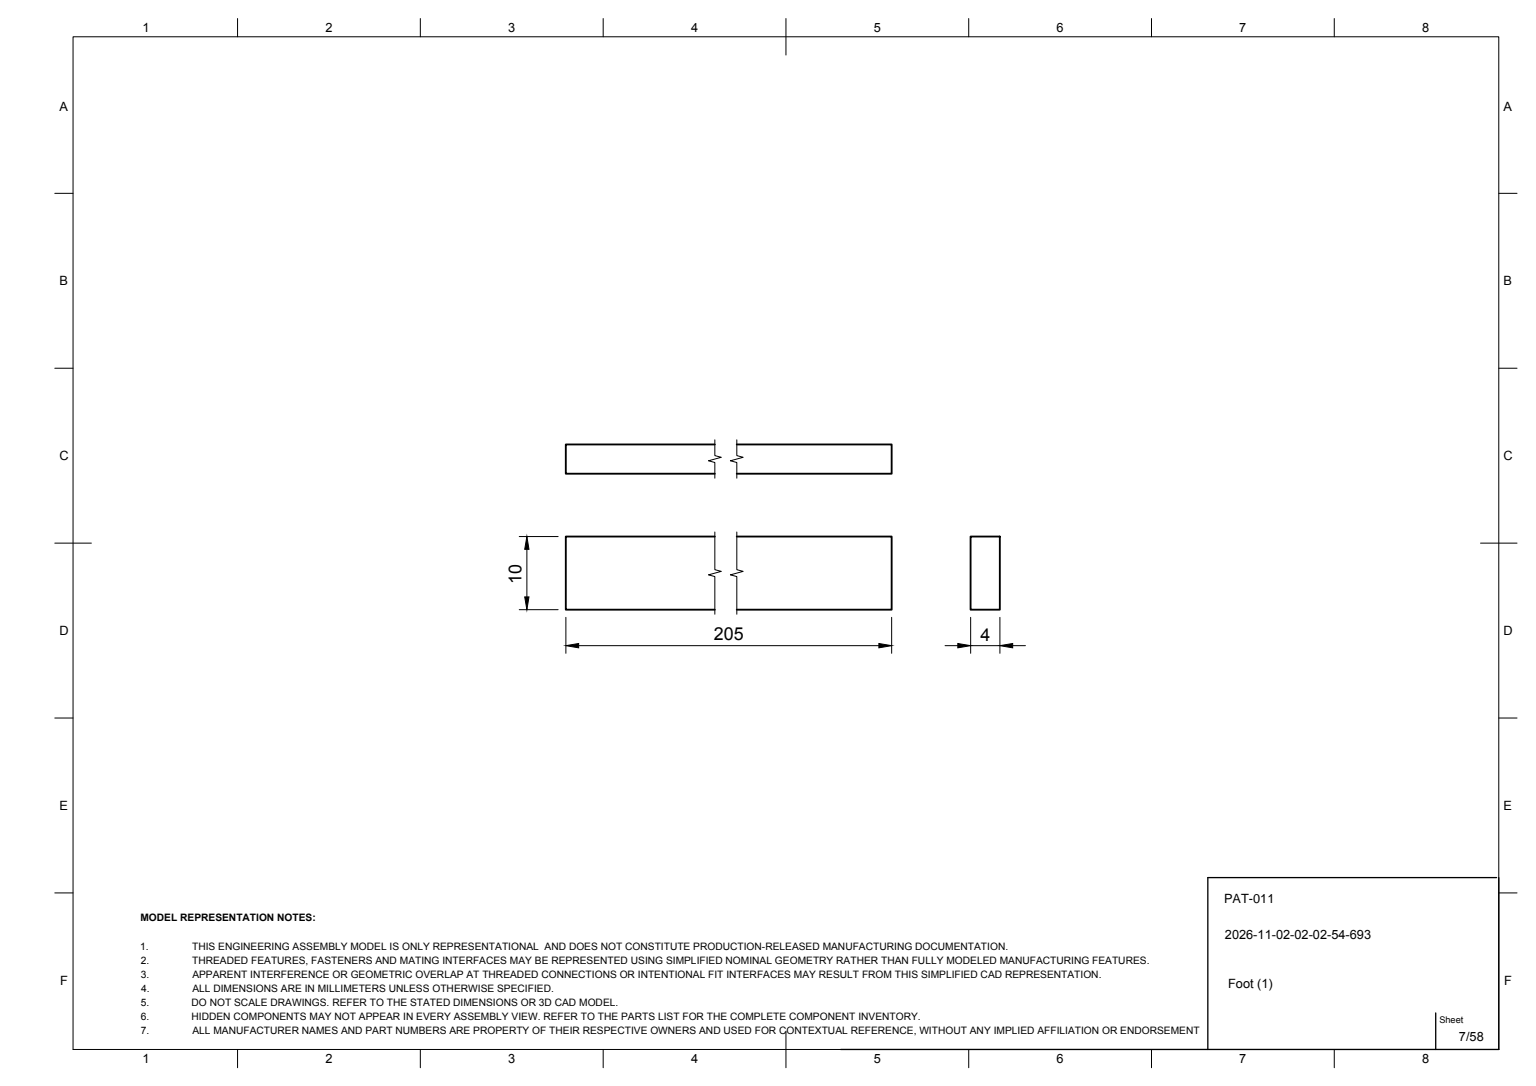
ISO-10303-21;
HEADER;
/* Generated by software containing ST-Developer
 * from STEP Tools, Inc. (www.steptools.com) 
 */

FILE_DESCRIPTION(
/* description */ ('Belt tension measurement rig'),
/* implementation_level */ '2;1');

FILE_NAME(
/* name */ 'Foot (1).step',
/* time_stamp */ '2026-10-28T03:24:44-07:00',
/* author */ (''),
/* organization */ (''),
/* preprocessor_version */ 'ST-DEVELOPER v20.2',
/* originating_system */ 'Autodesk Translation Framework v15.17.0.0',
/* authorisation */ '');

FILE_SCHEMA (('AUTOMOTIVE_DESIGN { 1 0 10303 214 3 1 1 }'));
ENDSEC;

DATA;
#10=MECHANICAL_DESIGN_GEOMETRIC_PRESENTATION_REPRESENTATION('',(#694),#23587);
#584=SHAPE_REPRESENTATION_RELATIONSHIP('SRR','None',#23829,#639);
#639=ADVANCED_BREP_SHAPE_REPRESENTATION('',(#764),#23527);
#694=STYLED_ITEM('',(#24225),#764);
#764=MANIFOLD_SOLID_BREP('Body1',#12199);
#1063=PLANE('',#12949);
#1064=PLANE('',#12950);
#1065=PLANE('',#12951);
#1066=PLANE('',#12952);
#1067=PLANE('',#12953);
#1068=PLANE('',#12954);
#1392=FACE_OUTER_BOUND('',#2110,.T.);
#1393=FACE_OUTER_BOUND('',#2111,.T.);
#1394=FACE_OUTER_BOUND('',#2112,.T.);
#1395=FACE_OUTER_BOUND('',#2113,.T.);
#1396=FACE_OUTER_BOUND('',#2114,.T.);
#1397=FACE_OUTER_BOUND('',#2115,.T.);
#2110=EDGE_LOOP('',(#8070,#8071,#8072,#8073));
#2111=EDGE_LOOP('',(#8074,#8075,#8076,#8077));
#2112=EDGE_LOOP('',(#8078,#8079,#8080,#8081));
#2113=EDGE_LOOP('',(#8082,#8083,#8084,#8085));
#2114=EDGE_LOOP('',(#8086,#8087,#8088,#8089));
#2115=EDGE_LOOP('',(#8090,#8091,#8092,#8093));
#3006=LINE('',#18708,#3757);
#3007=LINE('',#18710,#3758);
#3008=LINE('',#18712,#3759);
#3009=LINE('',#18713,#3760);
#3010=LINE('',#18716,#3761);
#3011=LINE('',#18718,#3762);
#3012=LINE('',#18719,#3763);
#3013=LINE('',#18722,#3764);
#3014=LINE('',#18724,#3765);
#3015=LINE('',#18725,#3766);
#3016=LINE('',#18727,#3767);
#3017=LINE('',#18728,#3768);
#3757=VECTOR('',#14703,1.);
#3758=VECTOR('',#14704,1.);
#3759=VECTOR('',#14705,1.);
#3760=VECTOR('',#14706,1.);
#3761=VECTOR('',#14709,1.);
#3762=VECTOR('',#14710,1.);
#3763=VECTOR('',#14711,1.);
#3764=VECTOR('',#14714,1.);
#3765=VECTOR('',#14715,1.);
#3766=VECTOR('',#14716,1.);
#3767=VECTOR('',#14719,1.);
#3768=VECTOR('',#14720,1.);
#5282=VERTEX_POINT('',#18706);
#5283=VERTEX_POINT('',#18707);
#5284=VERTEX_POINT('',#18709);
#5285=VERTEX_POINT('',#18711);
#5286=VERTEX_POINT('',#18715);
#5287=VERTEX_POINT('',#18717);
#5288=VERTEX_POINT('',#18721);
#5289=VERTEX_POINT('',#18723);
#6394=EDGE_CURVE('',#5282,#5283,#3006,.T.);
#6395=EDGE_CURVE('',#5283,#5284,#3007,.T.);
#6396=EDGE_CURVE('',#5285,#5284,#3008,.T.);
#6397=EDGE_CURVE('',#5282,#5285,#3009,.T.);
#6398=EDGE_CURVE('',#5286,#5282,#3010,.T.);
#6399=EDGE_CURVE('',#5287,#5285,#3011,.T.);
#6400=EDGE_CURVE('',#5286,#5287,#3012,.T.);
#6401=EDGE_CURVE('',#5288,#5286,#3013,.T.);
#6402=EDGE_CURVE('',#5289,#5287,#3014,.T.);
#6403=EDGE_CURVE('',#5288,#5289,#3015,.T.);
#6404=EDGE_CURVE('',#5283,#5288,#3016,.T.);
#6405=EDGE_CURVE('',#5284,#5289,#3017,.T.);
#8070=ORIENTED_EDGE('',*,*,#6394,.T.);
#8071=ORIENTED_EDGE('',*,*,#6395,.T.);
#8072=ORIENTED_EDGE('',*,*,#6396,.F.);
#8073=ORIENTED_EDGE('',*,*,#6397,.F.);
#8074=ORIENTED_EDGE('',*,*,#6398,.T.);
#8075=ORIENTED_EDGE('',*,*,#6397,.T.);
#8076=ORIENTED_EDGE('',*,*,#6399,.F.);
#8077=ORIENTED_EDGE('',*,*,#6400,.F.);
#8078=ORIENTED_EDGE('',*,*,#6401,.T.);
#8079=ORIENTED_EDGE('',*,*,#6400,.T.);
#8080=ORIENTED_EDGE('',*,*,#6402,.F.);
#8081=ORIENTED_EDGE('',*,*,#6403,.F.);
#8082=ORIENTED_EDGE('',*,*,#6404,.T.);
#8083=ORIENTED_EDGE('',*,*,#6403,.T.);
#8084=ORIENTED_EDGE('',*,*,#6405,.F.);
#8085=ORIENTED_EDGE('',*,*,#6395,.F.);
#8086=ORIENTED_EDGE('',*,*,#6405,.T.);
#8087=ORIENTED_EDGE('',*,*,#6402,.T.);
#8088=ORIENTED_EDGE('',*,*,#6399,.T.);
#8089=ORIENTED_EDGE('',*,*,#6396,.T.);
#8090=ORIENTED_EDGE('',*,*,#6404,.F.);
#8091=ORIENTED_EDGE('',*,*,#6394,.F.);
#8092=ORIENTED_EDGE('',*,*,#6398,.F.);
#8093=ORIENTED_EDGE('',*,*,#6401,.F.);
#11533=ADVANCED_FACE('',(#1392),#1063,.T.);
#11534=ADVANCED_FACE('',(#1393),#1064,.T.);
#11535=ADVANCED_FACE('',(#1394),#1065,.T.);
#11536=ADVANCED_FACE('',(#1395),#1066,.T.);
#11537=ADVANCED_FACE('',(#1396),#1067,.T.);
#11538=ADVANCED_FACE('',(#1397),#1068,.F.);
#12199=CLOSED_SHELL('',(#11533,#11534,#11535,#11536,#11537,#11538));
#12948=AXIS2_PLACEMENT_3D('',#18704,#14699,#14700);
#12949=AXIS2_PLACEMENT_3D('',#18705,#14701,#14702);
#12950=AXIS2_PLACEMENT_3D('',#18714,#14707,#14708);
#12951=AXIS2_PLACEMENT_3D('',#18720,#14712,#14713);
#12952=AXIS2_PLACEMENT_3D('',#18726,#14717,#14718);
#12953=AXIS2_PLACEMENT_3D('',#18729,#14721,#14722);
#12954=AXIS2_PLACEMENT_3D('',#18730,#14723,#14724);
#14699=DIRECTION('axis',(0.,0.,1.));
#14700=DIRECTION('refdir',(1.,0.,0.));
#14701=DIRECTION('center_axis',(0.,1.,0.));
#14702=DIRECTION('ref_axis',(-1.,0.,0.));
#14703=DIRECTION('',(-1.,0.,0.));
#14704=DIRECTION('',(0.,0.,1.));
#14705=DIRECTION('',(-1.,0.,0.));
#14706=DIRECTION('',(0.,0.,1.));
#14707=DIRECTION('center_axis',(1.,0.,0.));
#14708=DIRECTION('ref_axis',(0.,1.,0.));
#14709=DIRECTION('',(0.,1.,0.));
#14710=DIRECTION('',(0.,1.,0.));
#14711=DIRECTION('',(0.,0.,1.));
#14712=DIRECTION('center_axis',(0.,-1.,0.));
#14713=DIRECTION('ref_axis',(1.,0.,0.));
#14714=DIRECTION('',(1.,0.,0.));
#14715=DIRECTION('',(1.,0.,0.));
#14716=DIRECTION('',(0.,0.,1.));
#14717=DIRECTION('center_axis',(-1.,0.,0.));
#14718=DIRECTION('ref_axis',(0.,-1.,0.));
#14719=DIRECTION('',(0.,-1.,0.));
#14720=DIRECTION('',(0.,-1.,0.));
#14721=DIRECTION('center_axis',(0.,0.,1.));
#14722=DIRECTION('ref_axis',(1.,0.,0.));
#14723=DIRECTION('center_axis',(0.,0.,1.));
#14724=DIRECTION('ref_axis',(1.,0.,0.));
#18704=CARTESIAN_POINT('',(0.,0.,0.));
#18705=CARTESIAN_POINT('Origin',(25.,14.,-1.6));
#18706=CARTESIAN_POINT('',(25.,14.,-1.6));
#18707=CARTESIAN_POINT('',(24.,14.,-1.6));
#18708=CARTESIAN_POINT('',(25.,14.,-1.6));
#18709=CARTESIAN_POINT('',(24.,14.,-1.2));
#18710=CARTESIAN_POINT('',(24.,14.,-1.6));
#18711=CARTESIAN_POINT('',(25.,14.,-1.2));
#18712=CARTESIAN_POINT('',(25.,14.,-1.2));
#18713=CARTESIAN_POINT('',(25.,14.,-1.6));
#18714=CARTESIAN_POINT('Origin',(25.,-6.5,-1.6));
#18715=CARTESIAN_POINT('',(25.,-6.5,-1.6));
#18716=CARTESIAN_POINT('',(25.,-6.5,-1.6));
#18717=CARTESIAN_POINT('',(25.,-6.5,-1.2));
#18718=CARTESIAN_POINT('',(25.,-6.5,-1.2));
#18719=CARTESIAN_POINT('',(25.,-6.5,-1.6));
#18720=CARTESIAN_POINT('Origin',(24.,-6.5,-1.6));
#18721=CARTESIAN_POINT('',(24.,-6.5,-1.6));
#18722=CARTESIAN_POINT('',(24.,-6.5,-1.6));
#18723=CARTESIAN_POINT('',(24.,-6.5,-1.2));
#18724=CARTESIAN_POINT('',(24.,-6.5,-1.2));
#18725=CARTESIAN_POINT('',(24.,-6.5,-1.6));
#18726=CARTESIAN_POINT('Origin',(24.,14.,-1.6));
#18727=CARTESIAN_POINT('',(24.,14.,-1.6));
#18728=CARTESIAN_POINT('',(24.,14.,-1.2));
#18729=CARTESIAN_POINT('Origin',(24.5,3.75,-1.2));
#18730=CARTESIAN_POINT('Origin',(24.5,3.75,-1.6));
#23462=UNCERTAINTY_MEASURE_WITH_UNIT(LENGTH_MEASURE(0.001),#23588,
'DISTANCE_ACCURACY_VALUE',
'Maximum model space distance between geometric entities at asserted c
onnectivities');
#23522=UNCERTAINTY_MEASURE_WITH_UNIT(LENGTH_MEASURE(0.001),#23588,
'DISTANCE_ACCURACY_VALUE',
'Maximum model space distance between geometric entities at asserted c
onnectivities');
#23527=(
GEOMETRIC_REPRESENTATION_CONTEXT(3)
GLOBAL_UNCERTAINTY_ASSIGNED_CONTEXT((#23462))
GLOBAL_UNIT_ASSIGNED_CONTEXT((#23588,#23590,#23591))
REPRESENTATION_CONTEXT('','3D')
);
#23587=(
GEOMETRIC_REPRESENTATION_CONTEXT(3)
GLOBAL_UNCERTAINTY_ASSIGNED_CONTEXT((#23522))
GLOBAL_UNIT_ASSIGNED_CONTEXT((#23588,#23590,#23591))
REPRESENTATION_CONTEXT('','3D')
);
#23588=(
LENGTH_UNIT()
NAMED_UNIT(*)
SI_UNIT(.CENTI.,.METRE.)
);
#23590=(
NAMED_UNIT(*)
PLANE_ANGLE_UNIT()
SI_UNIT($,.RADIAN.)
);
#23591=(
NAMED_UNIT(*)
SI_UNIT($,.STERADIAN.)
SOLID_ANGLE_UNIT()
);
#23596=SHAPE_DEFINITION_REPRESENTATION(#23660,#23829);
#23660=PRODUCT_DEFINITION_SHAPE('',$,#23894);
#23829=SHAPE_REPRESENTATION('',(#12948),#23527);
#23889=PRODUCT_DEFINITION_CONTEXT('part definition',#24083,'design');
#23894=PRODUCT_DEFINITION('Foot (1)','Foot (1)',#23958,#23889);
#23958=PRODUCT_DEFINITION_FORMATION('',$,#24089);
#24083=APPLICATION_CONTEXT(
'Core Data for Automotive Mechanical Design Process');
#24084=PRODUCT_CONTEXT('part definition',#24083,'mechanical');
#24089=PRODUCT('Foot (1)','Foot (1)','Foot (1)',(#24084));
#24219=COLOUR_RGB('Off White',0.89,0.88,0.83);
#24220=FILL_AREA_STYLE_COLOUR('',#24219);
#24221=FILL_AREA_STYLE('',(#24220));
#24222=SURFACE_STYLE_FILL_AREA(#24221);
#24223=SURFACE_SIDE_STYLE('',(#24222));
#24224=SURFACE_STYLE_USAGE(.BOTH.,#24223);
#24225=PRESENTATION_STYLE_ASSIGNMENT((#24224));
ENDSEC;
END-ISO-10303-21;
